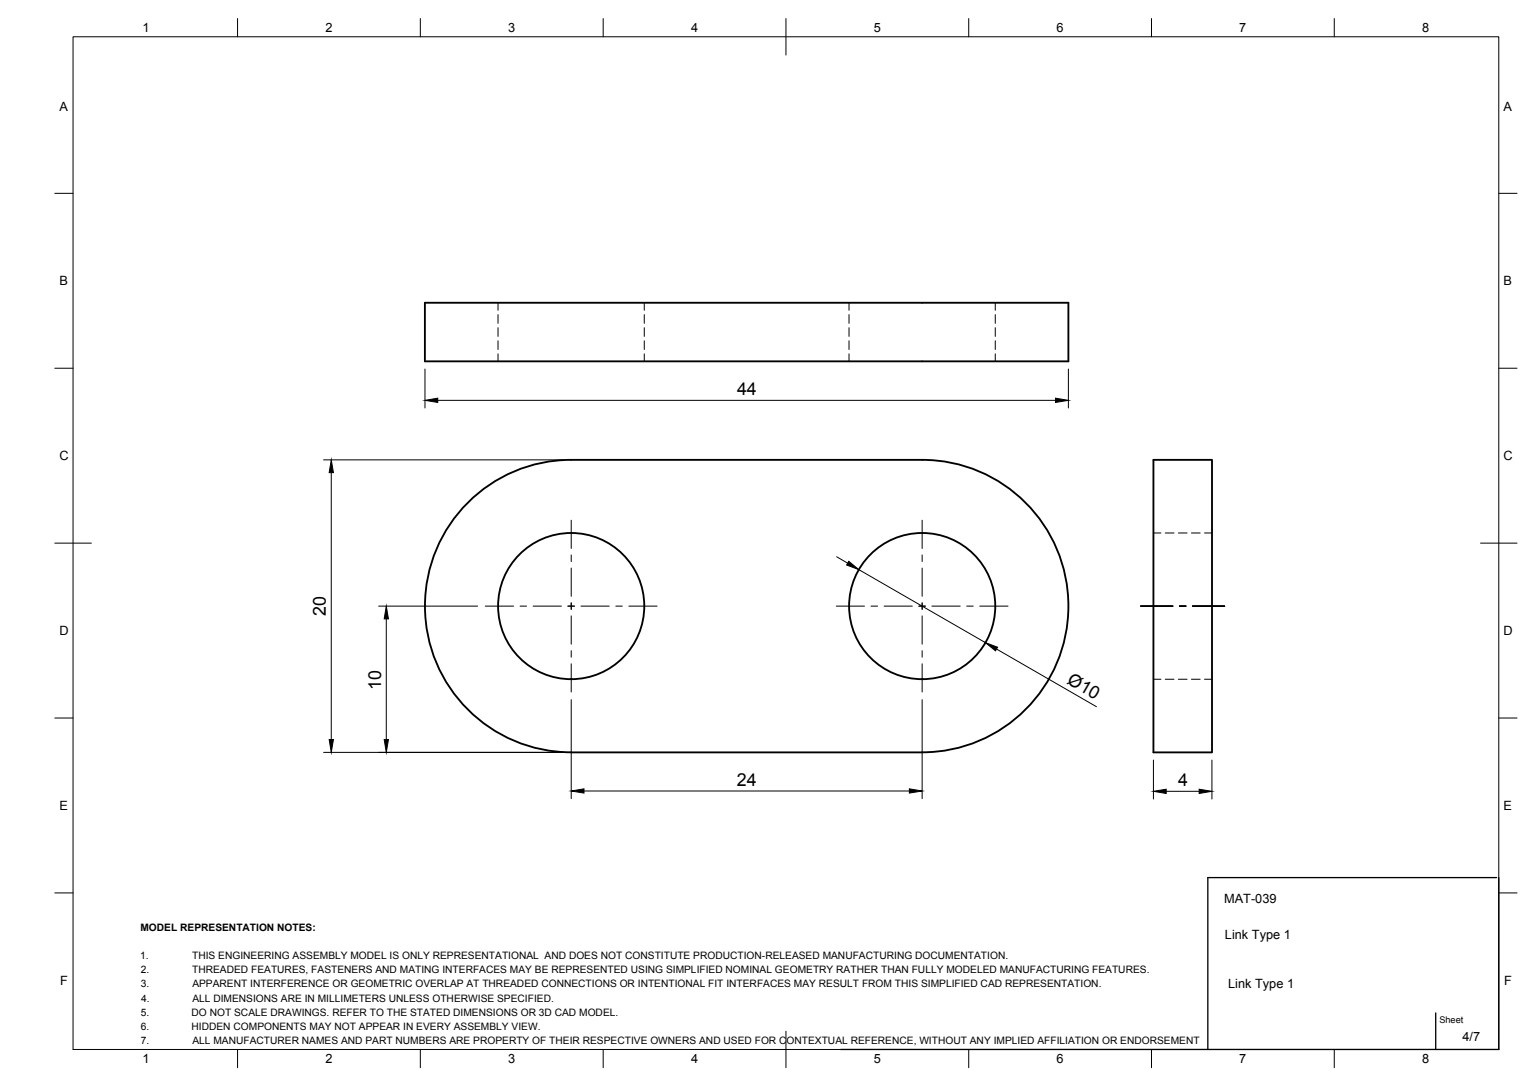
ISO-10303-21;
HEADER;
/* Generated by software containing ST-Developer
 * from STEP Tools, Inc. (www.steptools.com) 
 */

FILE_DESCRIPTION(
/* description */ ('STEP AP214'),
/* implementation_level */ '2;1');

FILE_NAME(
/* name */ 'Link Type 1.step',
/* time_stamp */ '2026-11-14T21:46:24-08:00',
/* author */ (''),
/* organization */ (''),
/* preprocessor_version */ 'ST-DEVELOPER v20.2',
/* originating_system */ 'Autodesk Translation Framework v15.17.0.0',
/* authorisation */ '');

FILE_SCHEMA (('AUTOMOTIVE_DESIGN { 1 0 10303 214 3 1 1 }'));
ENDSEC;

DATA;
#10=MECHANICAL_DESIGN_GEOMETRIC_PRESENTATION_REPRESENTATION('',(#92),#7783);
#78=SHAPE_REPRESENTATION_RELATIONSHIP('SRR','None',#7823,#85);
#85=ADVANCED_BREP_SHAPE_REPRESENTATION('',(#99),#7779);
#92=STYLED_ITEM('',(#7870),#99);
#99=MANIFOLD_SOLID_BREP('Body1',#4167);
#137=FACE_BOUND('',#1483,.T.);
#138=FACE_BOUND('',#1484,.T.);
#139=FACE_BOUND('',#1486,.T.);
#140=FACE_BOUND('',#1487,.T.);
#244=PLANE('',#4471);
#245=PLANE('',#4473);
#246=PLANE('',#4475);
#247=PLANE('',#4477);
#512=LINE('',#6635,#871);
#513=LINE('',#6641,#872);
#514=LINE('',#6648,#873);
#515=LINE('',#6651,#874);
#516=LINE('',#6654,#875);
#517=LINE('',#6657,#876);
#518=LINE('',#6660,#877);
#519=LINE('',#6663,#878);
#520=LINE('',#6665,#879);
#521=LINE('',#6667,#880);
#871=VECTOR('',#5365,5.);
#872=VECTOR('',#5372,5.);
#873=VECTOR('',#5379,1000.);
#874=VECTOR('',#5382,1000.);
#875=VECTOR('',#5385,1000.);
#876=VECTOR('',#5388,1000.);
#877=VECTOR('',#5391,1000.);
#878=VECTOR('',#5394,1000.);
#879=VECTOR('',#5397,1000.);
#880=VECTOR('',#5400,1000.);
#1041=CYLINDRICAL_SURFACE('',#4462,5.);
#1042=CYLINDRICAL_SURFACE('',#4465,5.);
#1043=CYLINDRICAL_SURFACE('',#4468,10.);
#1044=CYLINDRICAL_SURFACE('',#4476,10.);
#1211=FACE_OUTER_BOUND('',#1479,.T.);
#1212=FACE_OUTER_BOUND('',#1480,.T.);
#1213=FACE_OUTER_BOUND('',#1481,.T.);
#1214=FACE_OUTER_BOUND('',#1482,.T.);
#1215=FACE_OUTER_BOUND('',#1485,.T.);
#1216=FACE_OUTER_BOUND('',#1488,.T.);
#1217=FACE_OUTER_BOUND('',#1489,.T.);
#1218=FACE_OUTER_BOUND('',#1490,.T.);
#1479=EDGE_LOOP('',(#3366,#3367,#3368,#3369));
#1480=EDGE_LOOP('',(#3370,#3371,#3372,#3373));
#1481=EDGE_LOOP('',(#3374,#3375,#3376,#3377));
#1482=EDGE_LOOP('',(#3378,#3379,#3380,#3381));
#1483=EDGE_LOOP('',(#3382));
#1484=EDGE_LOOP('',(#3383));
#1485=EDGE_LOOP('',(#3384,#3385,#3386,#3387));
#1486=EDGE_LOOP('',(#3388));
#1487=EDGE_LOOP('',(#3389));
#1488=EDGE_LOOP('',(#3390,#3391,#3392,#3393));
#1489=EDGE_LOOP('',(#3394,#3395,#3396,#3397));
#1490=EDGE_LOOP('',(#3398,#3399,#3400,#3401));
#1700=CIRCLE('',#4463,5.);
#1701=CIRCLE('',#4464,5.);
#1702=CIRCLE('',#4466,5.);
#1703=CIRCLE('',#4467,5.);
#1704=CIRCLE('',#4469,10.);
#1705=CIRCLE('',#4470,10.);
#1706=CIRCLE('',#4472,10.);
#1707=CIRCLE('',#4474,10.);
#2020=VERTEX_POINT('',#6632);
#2021=VERTEX_POINT('',#6634);
#2022=VERTEX_POINT('',#6638);
#2023=VERTEX_POINT('',#6640);
#2024=VERTEX_POINT('',#6644);
#2025=VERTEX_POINT('',#6645);
#2026=VERTEX_POINT('',#6647);
#2027=VERTEX_POINT('',#6649);
#2028=VERTEX_POINT('',#6653);
#2029=VERTEX_POINT('',#6655);
#2030=VERTEX_POINT('',#6659);
#2031=VERTEX_POINT('',#6661);
#2490=EDGE_CURVE('',#2020,#2020,#1700,.T.);
#2491=EDGE_CURVE('',#2020,#2021,#512,.T.);
#2492=EDGE_CURVE('',#2021,#2021,#1701,.T.);
#2493=EDGE_CURVE('',#2022,#2022,#1702,.T.);
#2494=EDGE_CURVE('',#2022,#2023,#513,.T.);
#2495=EDGE_CURVE('',#2023,#2023,#1703,.T.);
#2496=EDGE_CURVE('',#2024,#2025,#1704,.T.);
#2497=EDGE_CURVE('',#2024,#2026,#514,.T.);
#2498=EDGE_CURVE('',#2026,#2027,#1705,.T.);
#2499=EDGE_CURVE('',#2025,#2027,#515,.T.);
#2500=EDGE_CURVE('',#2025,#2028,#516,.T.);
#2501=EDGE_CURVE('',#2028,#2029,#1706,.T.);
#2502=EDGE_CURVE('',#2029,#2024,#517,.T.);
#2503=EDGE_CURVE('',#2030,#2026,#518,.T.);
#2504=EDGE_CURVE('',#2031,#2030,#1707,.T.);
#2505=EDGE_CURVE('',#2027,#2031,#519,.T.);
#2506=EDGE_CURVE('',#2028,#2031,#520,.T.);
#2507=EDGE_CURVE('',#2029,#2030,#521,.T.);
#3366=ORIENTED_EDGE('',*,*,#2490,.T.);
#3367=ORIENTED_EDGE('',*,*,#2491,.T.);
#3368=ORIENTED_EDGE('',*,*,#2492,.F.);
#3369=ORIENTED_EDGE('',*,*,#2491,.F.);
#3370=ORIENTED_EDGE('',*,*,#2493,.T.);
#3371=ORIENTED_EDGE('',*,*,#2494,.T.);
#3372=ORIENTED_EDGE('',*,*,#2495,.F.);
#3373=ORIENTED_EDGE('',*,*,#2494,.F.);
#3374=ORIENTED_EDGE('',*,*,#2496,.F.);
#3375=ORIENTED_EDGE('',*,*,#2497,.T.);
#3376=ORIENTED_EDGE('',*,*,#2498,.T.);
#3377=ORIENTED_EDGE('',*,*,#2499,.F.);
#3378=ORIENTED_EDGE('',*,*,#2496,.T.);
#3379=ORIENTED_EDGE('',*,*,#2500,.T.);
#3380=ORIENTED_EDGE('',*,*,#2501,.T.);
#3381=ORIENTED_EDGE('',*,*,#2502,.T.);
#3382=ORIENTED_EDGE('',*,*,#2490,.F.);
#3383=ORIENTED_EDGE('',*,*,#2493,.F.);
#3384=ORIENTED_EDGE('',*,*,#2498,.F.);
#3385=ORIENTED_EDGE('',*,*,#2503,.F.);
#3386=ORIENTED_EDGE('',*,*,#2504,.F.);
#3387=ORIENTED_EDGE('',*,*,#2505,.F.);
#3388=ORIENTED_EDGE('',*,*,#2492,.T.);
#3389=ORIENTED_EDGE('',*,*,#2495,.T.);
#3390=ORIENTED_EDGE('',*,*,#2505,.T.);
#3391=ORIENTED_EDGE('',*,*,#2506,.F.);
#3392=ORIENTED_EDGE('',*,*,#2500,.F.);
#3393=ORIENTED_EDGE('',*,*,#2499,.T.);
#3394=ORIENTED_EDGE('',*,*,#2504,.T.);
#3395=ORIENTED_EDGE('',*,*,#2507,.F.);
#3396=ORIENTED_EDGE('',*,*,#2501,.F.);
#3397=ORIENTED_EDGE('',*,*,#2506,.T.);
#3398=ORIENTED_EDGE('',*,*,#2503,.T.);
#3399=ORIENTED_EDGE('',*,*,#2497,.F.);
#3400=ORIENTED_EDGE('',*,*,#2502,.F.);
#3401=ORIENTED_EDGE('',*,*,#2507,.T.);
#4046=ADVANCED_FACE('',(#1211),#1041,.F.);
#4047=ADVANCED_FACE('',(#1212),#1042,.F.);
#4048=ADVANCED_FACE('',(#1213),#1043,.T.);
#4049=ADVANCED_FACE('',(#1214,#137,#138),#244,.T.);
#4050=ADVANCED_FACE('',(#1215,#139,#140),#245,.F.);
#4051=ADVANCED_FACE('',(#1216),#246,.F.);
#4052=ADVANCED_FACE('',(#1217),#1044,.T.);
#4053=ADVANCED_FACE('',(#1218),#247,.F.);
#4167=CLOSED_SHELL('',(#4046,#4047,#4048,#4049,#4050,#4051,#4052,#4053));
#4461=AXIS2_PLACEMENT_3D('',#6630,#5359,#5360);
#4462=AXIS2_PLACEMENT_3D('',#6631,#5361,#5362);
#4463=AXIS2_PLACEMENT_3D('',#6633,#5363,#5364);
#4464=AXIS2_PLACEMENT_3D('',#6636,#5366,#5367);
#4465=AXIS2_PLACEMENT_3D('',#6637,#5368,#5369);
#4466=AXIS2_PLACEMENT_3D('',#6639,#5370,#5371);
#4467=AXIS2_PLACEMENT_3D('',#6642,#5373,#5374);
#4468=AXIS2_PLACEMENT_3D('',#6643,#5375,#5376);
#4469=AXIS2_PLACEMENT_3D('',#6646,#5377,#5378);
#4470=AXIS2_PLACEMENT_3D('',#6650,#5380,#5381);
#4471=AXIS2_PLACEMENT_3D('',#6652,#5383,#5384);
#4472=AXIS2_PLACEMENT_3D('',#6656,#5386,#5387);
#4473=AXIS2_PLACEMENT_3D('',#6658,#5389,#5390);
#4474=AXIS2_PLACEMENT_3D('',#6662,#5392,#5393);
#4475=AXIS2_PLACEMENT_3D('',#6664,#5395,#5396);
#4476=AXIS2_PLACEMENT_3D('',#6666,#5398,#5399);
#4477=AXIS2_PLACEMENT_3D('',#6668,#5401,#5402);
#5359=DIRECTION('axis',(0.,0.,1.));
#5360=DIRECTION('refdir',(1.,0.,0.));
#5361=DIRECTION('center_axis',(0.,0.,-1.));
#5362=DIRECTION('ref_axis',(-1.,0.,0.));
#5363=DIRECTION('center_axis',(0.,0.,1.));
#5364=DIRECTION('ref_axis',(1.,0.,0.));
#5365=DIRECTION('',(0.,0.,-1.));
#5366=DIRECTION('center_axis',(0.,0.,1.));
#5367=DIRECTION('ref_axis',(1.,0.,0.));
#5368=DIRECTION('center_axis',(0.,0.,-1.));
#5369=DIRECTION('ref_axis',(-1.,0.,0.));
#5370=DIRECTION('center_axis',(0.,0.,1.));
#5371=DIRECTION('ref_axis',(1.,0.,0.));
#5372=DIRECTION('',(0.,0.,-1.));
#5373=DIRECTION('center_axis',(0.,0.,1.));
#5374=DIRECTION('ref_axis',(1.,0.,0.));
#5375=DIRECTION('center_axis',(0.,0.,-1.));
#5376=DIRECTION('ref_axis',(-1.,0.,0.));
#5377=DIRECTION('center_axis',(0.,0.,1.));
#5378=DIRECTION('ref_axis',(1.,0.,0.));
#5379=DIRECTION('',(0.,0.,-1.));
#5380=DIRECTION('center_axis',(0.,0.,1.));
#5381=DIRECTION('ref_axis',(1.,0.,0.));
#5382=DIRECTION('',(0.,0.,-1.));
#5383=DIRECTION('center_axis',(0.,0.,1.));
#5384=DIRECTION('ref_axis',(1.,0.,0.));
#5385=DIRECTION('',(1.,1.44560289664734E-16,0.));
#5386=DIRECTION('center_axis',(0.,0.,1.));
#5387=DIRECTION('ref_axis',(-1.,0.,0.));
#5388=DIRECTION('',(-1.,0.,0.));
#5389=DIRECTION('center_axis',(0.,0.,1.));
#5390=DIRECTION('ref_axis',(1.,0.,0.));
#5391=DIRECTION('',(-1.,0.,0.));
#5392=DIRECTION('center_axis',(0.,0.,1.));
#5393=DIRECTION('ref_axis',(-1.,0.,0.));
#5394=DIRECTION('',(1.,1.44560289664734E-16,0.));
#5395=DIRECTION('center_axis',(-1.44560289664734E-16,1.,0.));
#5396=DIRECTION('ref_axis',(-1.,-1.44560289664734E-16,0.));
#5397=DIRECTION('',(0.,0.,-1.));
#5398=DIRECTION('center_axis',(0.,0.,-1.));
#5399=DIRECTION('ref_axis',(1.,1.22464679914735E-16,0.));
#5400=DIRECTION('',(0.,0.,-1.));
#5401=DIRECTION('center_axis',(0.,-1.,0.));
#5402=DIRECTION('ref_axis',(0.,0.,-1.));
#6630=CARTESIAN_POINT('',(0.,0.,0.));
#6631=CARTESIAN_POINT('Origin',(24.,0.,2.));
#6632=CARTESIAN_POINT('',(29.,-6.12323399573677E-16,2.));
#6633=CARTESIAN_POINT('Origin',(24.,0.,2.));
#6634=CARTESIAN_POINT('',(29.,-6.12323399573677E-16,-2.));
#6635=CARTESIAN_POINT('',(29.,-6.12323399573677E-16,2.));
#6636=CARTESIAN_POINT('Origin',(24.,0.,-2.));
#6637=CARTESIAN_POINT('Origin',(0.,0.,2.));
#6638=CARTESIAN_POINT('',(5.,-6.12323399573677E-16,2.));
#6639=CARTESIAN_POINT('Origin',(0.,0.,2.));
#6640=CARTESIAN_POINT('',(5.,-6.12323399573677E-16,-2.));
#6641=CARTESIAN_POINT('',(5.,-6.12323399573677E-16,2.));
#6642=CARTESIAN_POINT('Origin',(0.,0.,-2.));
#6643=CARTESIAN_POINT('Origin',(0.,0.,2.));
#6644=CARTESIAN_POINT('',(0.,10.,2.));
#6645=CARTESIAN_POINT('',(1.22460635382238E-15,-10.,2.));
#6646=CARTESIAN_POINT('Origin',(0.,0.,2.));
#6647=CARTESIAN_POINT('',(0.,10.,-2.));
#6648=CARTESIAN_POINT('',(0.,10.,2.));
#6649=CARTESIAN_POINT('',(1.22460635382238E-15,-10.,-2.));
#6650=CARTESIAN_POINT('Origin',(0.,0.,-2.));
#6651=CARTESIAN_POINT('',(1.22460635382238E-15,-10.,2.));
#6652=CARTESIAN_POINT('Origin',(0.,0.,2.));
#6653=CARTESIAN_POINT('',(24.,-10.,2.));
#6654=CARTESIAN_POINT('',(24.,-10.,2.));
#6655=CARTESIAN_POINT('',(24.,10.,2.));
#6656=CARTESIAN_POINT('Origin',(24.,0.,2.));
#6657=CARTESIAN_POINT('',(0.,10.,2.));
#6658=CARTESIAN_POINT('Origin',(0.,0.,-2.));
#6659=CARTESIAN_POINT('',(24.,10.,-2.));
#6660=CARTESIAN_POINT('',(0.,10.,-2.));
#6661=CARTESIAN_POINT('',(24.,-10.,-2.));
#6662=CARTESIAN_POINT('Origin',(24.,0.,-2.));
#6663=CARTESIAN_POINT('',(24.,-10.,-2.));
#6664=CARTESIAN_POINT('Origin',(24.,-10.,2.));
#6665=CARTESIAN_POINT('',(24.,-10.,2.));
#6666=CARTESIAN_POINT('Origin',(24.,0.,2.));
#6667=CARTESIAN_POINT('',(24.,10.,2.));
#6668=CARTESIAN_POINT('Origin',(0.,10.,2.));
#7769=UNCERTAINTY_MEASURE_WITH_UNIT(LENGTH_MEASURE(0.01),#7784,
'DISTANCE_ACCURACY_VALUE',
'Maximum model space distance between geometric entities at asserted c
onnectivities');
#7773=UNCERTAINTY_MEASURE_WITH_UNIT(LENGTH_MEASURE(0.01),#7784,
'DISTANCE_ACCURACY_VALUE',
'Maximum model space distance between geometric entities at asserted c
onnectivities');
#7779=(
GEOMETRIC_REPRESENTATION_CONTEXT(3)
GLOBAL_UNCERTAINTY_ASSIGNED_CONTEXT((#7769))
GLOBAL_UNIT_ASSIGNED_CONTEXT((#7784,#7786,#7787))
REPRESENTATION_CONTEXT('','3D')
);
#7783=(
GEOMETRIC_REPRESENTATION_CONTEXT(3)
GLOBAL_UNCERTAINTY_ASSIGNED_CONTEXT((#7773))
GLOBAL_UNIT_ASSIGNED_CONTEXT((#7784,#7786,#7787))
REPRESENTATION_CONTEXT('','3D')
);
#7784=(
LENGTH_UNIT()
NAMED_UNIT(*)
SI_UNIT(.MILLI.,.METRE.)
);
#7786=(
NAMED_UNIT(*)
PLANE_ANGLE_UNIT()
SI_UNIT($,.RADIAN.)
);
#7787=(
NAMED_UNIT(*)
SI_UNIT($,.STERADIAN.)
SOLID_ANGLE_UNIT()
);
#7793=SHAPE_DEFINITION_REPRESENTATION(#7803,#7823);
#7803=PRODUCT_DEFINITION_SHAPE('',$,#7833);
#7823=SHAPE_REPRESENTATION('',(#4461),#7779);
#7827=PRODUCT_DEFINITION_CONTEXT('part definition',#7856,'design');
#7833=PRODUCT_DEFINITION('Link Type 1','Link Type 1',#7842,#7827);
#7842=PRODUCT_DEFINITION_FORMATION('',$,#7863);
#7856=APPLICATION_CONTEXT(
'Core Data for Automotive Mechanical Design Process');
#7857=PRODUCT_CONTEXT('part definition',#7856,'mechanical');
#7863=PRODUCT('Link Type 1','Link Type 1',$,(#7857));
#7870=PRESENTATION_STYLE_ASSIGNMENT((#7875));
#7875=SURFACE_STYLE_USAGE(.BOTH.,#7880);
#7880=SURFACE_SIDE_STYLE('',(#7885));
#7885=SURFACE_STYLE_FILL_AREA(#7890);
#7890=FILL_AREA_STYLE('Opaque(97,158,199)',(#7895));
#7895=FILL_AREA_STYLE_COLOUR('Opaque(97,158,199)',#7900);
#7900=COLOUR_RGB('Opaque(97,158,199)',0.380392156862745,0.619607843137255,
0.780392156862745);
ENDSEC;
END-ISO-10303-21;
